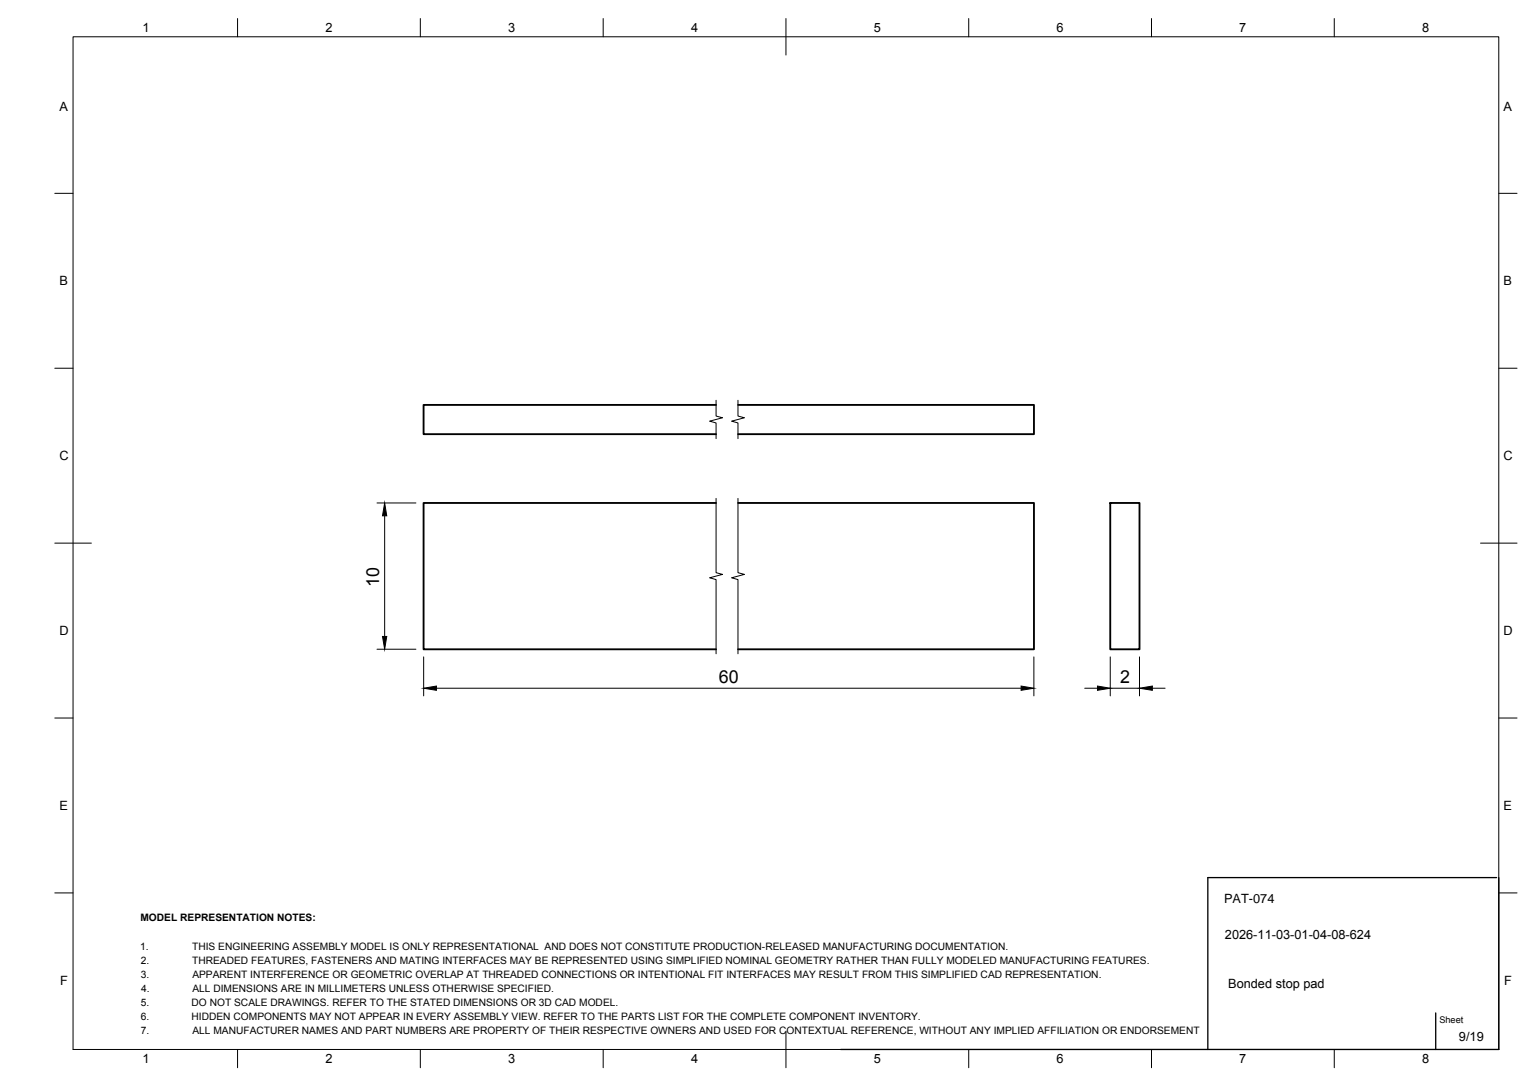
ISO-10303-21;
HEADER;
/* Generated by software containing ST-Developer
 * from STEP Tools, Inc. (www.steptools.com) 
 */

FILE_DESCRIPTION(
/* description */ ('Manual rail carriage with stops'),
/* implementation_level */ '2;1');

FILE_NAME(
/* name */ 'Bonded stop pad.step',
/* time_stamp */ '2026-10-27T18:54:27-07:00',
/* author */ (''),
/* organization */ (''),
/* preprocessor_version */ 'ST-DEVELOPER v20.2',
/* originating_system */ 'Autodesk Translation Framework v15.17.0.0',
/* authorisation */ '');

FILE_SCHEMA (('AUTOMOTIVE_DESIGN { 1 0 10303 214 3 1 1 }'));
ENDSEC;

DATA;
#10=MECHANICAL_DESIGN_GEOMETRIC_PRESENTATION_REPRESENTATION('',(#280),#8499);
#244=SHAPE_REPRESENTATION_RELATIONSHIP('SRR','None',#8607,#262);
#262=ADVANCED_BREP_SHAPE_REPRESENTATION('',(#296),#8486);
#280=STYLED_ITEM('',(#8802),#296);
#296=MANIFOLD_SOLID_BREP('Body1',#4950);
#493=PLANE('',#5399);
#494=PLANE('',#5400);
#495=PLANE('',#5401);
#496=PLANE('',#5402);
#497=PLANE('',#5403);
#498=PLANE('',#5404);
#729=FACE_OUTER_BOUND('',#1045,.T.);
#730=FACE_OUTER_BOUND('',#1046,.T.);
#731=FACE_OUTER_BOUND('',#1047,.T.);
#732=FACE_OUTER_BOUND('',#1048,.T.);
#733=FACE_OUTER_BOUND('',#1049,.T.);
#734=FACE_OUTER_BOUND('',#1050,.T.);
#1045=EDGE_LOOP('',(#4108,#4109,#4110,#4111));
#1046=EDGE_LOOP('',(#4112,#4113,#4114,#4115));
#1047=EDGE_LOOP('',(#4116,#4117,#4118,#4119));
#1048=EDGE_LOOP('',(#4120,#4121,#4122,#4123));
#1049=EDGE_LOOP('',(#4124,#4125,#4126,#4127));
#1050=EDGE_LOOP('',(#4128,#4129,#4130,#4131));
#1481=LINE('',#7855,#1981);
#1482=LINE('',#7857,#1982);
#1483=LINE('',#7859,#1983);
#1484=LINE('',#7860,#1984);
#1485=LINE('',#7863,#1985);
#1486=LINE('',#7865,#1986);
#1487=LINE('',#7866,#1987);
#1488=LINE('',#7869,#1988);
#1489=LINE('',#7871,#1989);
#1490=LINE('',#7872,#1990);
#1491=LINE('',#7874,#1991);
#1492=LINE('',#7875,#1992);
#1981=VECTOR('',#6406,1.);
#1982=VECTOR('',#6407,1.);
#1983=VECTOR('',#6408,1.);
#1984=VECTOR('',#6409,1.);
#1985=VECTOR('',#6412,1.);
#1986=VECTOR('',#6413,1.);
#1987=VECTOR('',#6414,1.);
#1988=VECTOR('',#6417,1.);
#1989=VECTOR('',#6418,1.);
#1990=VECTOR('',#6419,1.);
#1991=VECTOR('',#6422,1.);
#1992=VECTOR('',#6423,1.);
#2559=VERTEX_POINT('',#7853);
#2560=VERTEX_POINT('',#7854);
#2561=VERTEX_POINT('',#7856);
#2562=VERTEX_POINT('',#7858);
#2563=VERTEX_POINT('',#7862);
#2564=VERTEX_POINT('',#7864);
#2565=VERTEX_POINT('',#7868);
#2566=VERTEX_POINT('',#7870);
#3102=EDGE_CURVE('',#2559,#2560,#1481,.T.);
#3103=EDGE_CURVE('',#2560,#2561,#1482,.T.);
#3104=EDGE_CURVE('',#2562,#2561,#1483,.T.);
#3105=EDGE_CURVE('',#2559,#2562,#1484,.T.);
#3106=EDGE_CURVE('',#2563,#2559,#1485,.T.);
#3107=EDGE_CURVE('',#2564,#2562,#1486,.T.);
#3108=EDGE_CURVE('',#2563,#2564,#1487,.T.);
#3109=EDGE_CURVE('',#2565,#2563,#1488,.T.);
#3110=EDGE_CURVE('',#2566,#2564,#1489,.T.);
#3111=EDGE_CURVE('',#2565,#2566,#1490,.T.);
#3112=EDGE_CURVE('',#2560,#2565,#1491,.T.);
#3113=EDGE_CURVE('',#2561,#2566,#1492,.T.);
#4108=ORIENTED_EDGE('',*,*,#3102,.T.);
#4109=ORIENTED_EDGE('',*,*,#3103,.T.);
#4110=ORIENTED_EDGE('',*,*,#3104,.F.);
#4111=ORIENTED_EDGE('',*,*,#3105,.F.);
#4112=ORIENTED_EDGE('',*,*,#3106,.T.);
#4113=ORIENTED_EDGE('',*,*,#3105,.T.);
#4114=ORIENTED_EDGE('',*,*,#3107,.F.);
#4115=ORIENTED_EDGE('',*,*,#3108,.F.);
#4116=ORIENTED_EDGE('',*,*,#3109,.T.);
#4117=ORIENTED_EDGE('',*,*,#3108,.T.);
#4118=ORIENTED_EDGE('',*,*,#3110,.F.);
#4119=ORIENTED_EDGE('',*,*,#3111,.F.);
#4120=ORIENTED_EDGE('',*,*,#3112,.T.);
#4121=ORIENTED_EDGE('',*,*,#3111,.T.);
#4122=ORIENTED_EDGE('',*,*,#3113,.F.);
#4123=ORIENTED_EDGE('',*,*,#3103,.F.);
#4124=ORIENTED_EDGE('',*,*,#3113,.T.);
#4125=ORIENTED_EDGE('',*,*,#3110,.T.);
#4126=ORIENTED_EDGE('',*,*,#3107,.T.);
#4127=ORIENTED_EDGE('',*,*,#3104,.T.);
#4128=ORIENTED_EDGE('',*,*,#3112,.F.);
#4129=ORIENTED_EDGE('',*,*,#3102,.F.);
#4130=ORIENTED_EDGE('',*,*,#3106,.F.);
#4131=ORIENTED_EDGE('',*,*,#3109,.F.);
#4828=ADVANCED_FACE('',(#729),#493,.T.);
#4829=ADVANCED_FACE('',(#730),#494,.T.);
#4830=ADVANCED_FACE('',(#731),#495,.T.);
#4831=ADVANCED_FACE('',(#732),#496,.T.);
#4832=ADVANCED_FACE('',(#733),#497,.T.);
#4833=ADVANCED_FACE('',(#734),#498,.F.);
#4950=CLOSED_SHELL('',(#4828,#4829,#4830,#4831,#4832,#4833));
#5398=AXIS2_PLACEMENT_3D('',#7851,#6402,#6403);
#5399=AXIS2_PLACEMENT_3D('',#7852,#6404,#6405);
#5400=AXIS2_PLACEMENT_3D('',#7861,#6410,#6411);
#5401=AXIS2_PLACEMENT_3D('',#7867,#6415,#6416);
#5402=AXIS2_PLACEMENT_3D('',#7873,#6420,#6421);
#5403=AXIS2_PLACEMENT_3D('',#7876,#6424,#6425);
#5404=AXIS2_PLACEMENT_3D('',#7877,#6426,#6427);
#6402=DIRECTION('axis',(0.,0.,1.));
#6403=DIRECTION('refdir',(1.,0.,0.));
#6404=DIRECTION('center_axis',(0.,1.,0.));
#6405=DIRECTION('ref_axis',(-1.,0.,0.));
#6406=DIRECTION('',(-1.,0.,0.));
#6407=DIRECTION('',(0.,0.,1.));
#6408=DIRECTION('',(-1.,0.,0.));
#6409=DIRECTION('',(0.,0.,1.));
#6410=DIRECTION('center_axis',(1.,0.,0.));
#6411=DIRECTION('ref_axis',(0.,1.,0.));
#6412=DIRECTION('',(0.,1.,0.));
#6413=DIRECTION('',(0.,1.,0.));
#6414=DIRECTION('',(0.,0.,1.));
#6415=DIRECTION('center_axis',(0.,-1.,0.));
#6416=DIRECTION('ref_axis',(1.,0.,0.));
#6417=DIRECTION('',(1.,0.,0.));
#6418=DIRECTION('',(1.,0.,0.));
#6419=DIRECTION('',(0.,0.,1.));
#6420=DIRECTION('center_axis',(-1.,0.,0.));
#6421=DIRECTION('ref_axis',(0.,-1.,0.));
#6422=DIRECTION('',(0.,-1.,0.));
#6423=DIRECTION('',(0.,-1.,0.));
#6424=DIRECTION('center_axis',(0.,0.,1.));
#6425=DIRECTION('ref_axis',(1.,0.,0.));
#6426=DIRECTION('center_axis',(0.,0.,1.));
#6427=DIRECTION('ref_axis',(1.,0.,0.));
#7851=CARTESIAN_POINT('',(0.,0.,0.));
#7852=CARTESIAN_POINT('Origin',(0.2,3.,5.2));
#7853=CARTESIAN_POINT('',(0.2,3.,5.2));
#7854=CARTESIAN_POINT('',(0.,3.,5.2));
#7855=CARTESIAN_POINT('',(0.2,3.,5.2));
#7856=CARTESIAN_POINT('',(0.,3.,6.2));
#7857=CARTESIAN_POINT('',(0.,3.,5.2));
#7858=CARTESIAN_POINT('',(0.2,3.,6.2));
#7859=CARTESIAN_POINT('',(0.2,3.,6.2));
#7860=CARTESIAN_POINT('',(0.2,3.,5.2));
#7861=CARTESIAN_POINT('Origin',(0.2,-3.,5.2));
#7862=CARTESIAN_POINT('',(0.2,-3.,5.2));
#7863=CARTESIAN_POINT('',(0.2,-3.,5.2));
#7864=CARTESIAN_POINT('',(0.2,-3.,6.2));
#7865=CARTESIAN_POINT('',(0.2,-3.,6.2));
#7866=CARTESIAN_POINT('',(0.2,-3.,5.2));
#7867=CARTESIAN_POINT('Origin',(0.,-3.,5.2));
#7868=CARTESIAN_POINT('',(0.,-3.,5.2));
#7869=CARTESIAN_POINT('',(0.,-3.,5.2));
#7870=CARTESIAN_POINT('',(0.,-3.,6.2));
#7871=CARTESIAN_POINT('',(0.,-3.,6.2));
#7872=CARTESIAN_POINT('',(0.,-3.,5.2));
#7873=CARTESIAN_POINT('Origin',(0.,3.,5.2));
#7874=CARTESIAN_POINT('',(0.,3.,5.2));
#7875=CARTESIAN_POINT('',(0.,3.,6.2));
#7876=CARTESIAN_POINT('Origin',(0.1,0.,6.2));
#7877=CARTESIAN_POINT('Origin',(0.1,0.,5.2));
#8463=UNCERTAINTY_MEASURE_WITH_UNIT(LENGTH_MEASURE(0.001),#8500,
'DISTANCE_ACCURACY_VALUE',
'Maximum model space distance between geometric entities at asserted c
onnectivities');
#8476=UNCERTAINTY_MEASURE_WITH_UNIT(LENGTH_MEASURE(0.001),#8500,
'DISTANCE_ACCURACY_VALUE',
'Maximum model space distance between geometric entities at asserted c
onnectivities');
#8486=(
GEOMETRIC_REPRESENTATION_CONTEXT(3)
GLOBAL_UNCERTAINTY_ASSIGNED_CONTEXT((#8463))
GLOBAL_UNIT_ASSIGNED_CONTEXT((#8500,#8502,#8503))
REPRESENTATION_CONTEXT('','3D')
);
#8499=(
GEOMETRIC_REPRESENTATION_CONTEXT(3)
GLOBAL_UNCERTAINTY_ASSIGNED_CONTEXT((#8476))
GLOBAL_UNIT_ASSIGNED_CONTEXT((#8500,#8502,#8503))
REPRESENTATION_CONTEXT('','3D')
);
#8500=(
LENGTH_UNIT()
NAMED_UNIT(*)
SI_UNIT(.CENTI.,.METRE.)
);
#8502=(
NAMED_UNIT(*)
PLANE_ANGLE_UNIT()
SI_UNIT($,.RADIAN.)
);
#8503=(
NAMED_UNIT(*)
SI_UNIT($,.STERADIAN.)
SOLID_ANGLE_UNIT()
);
#8513=SHAPE_DEFINITION_REPRESENTATION(#8535,#8607);
#8535=PRODUCT_DEFINITION_SHAPE('',$,#8630);
#8607=SHAPE_REPRESENTATION('',(#5398),#8486);
#8620=PRODUCT_DEFINITION_CONTEXT('part definition',#8688,'design');
#8630=PRODUCT_DEFINITION('Bonded stop pad','Bonded stop pad',#8652,#8620);
#8652=PRODUCT_DEFINITION_FORMATION('',$,#8699);
#8688=APPLICATION_CONTEXT(
'Core Data for Automotive Mechanical Design Process');
#8689=PRODUCT_CONTEXT('part definition',#8688,'mechanical');
#8699=PRODUCT('Bonded stop pad','Bonded stop pad','Bonded stop pad',(#8689));
#8796=COLOUR_RGB('Off White',0.89,0.88,0.83);
#8797=FILL_AREA_STYLE_COLOUR('',#8796);
#8798=FILL_AREA_STYLE('',(#8797));
#8799=SURFACE_STYLE_FILL_AREA(#8798);
#8800=SURFACE_SIDE_STYLE('',(#8799));
#8801=SURFACE_STYLE_USAGE(.BOTH.,#8800);
#8802=PRESENTATION_STYLE_ASSIGNMENT((#8801));
ENDSEC;
END-ISO-10303-21;
